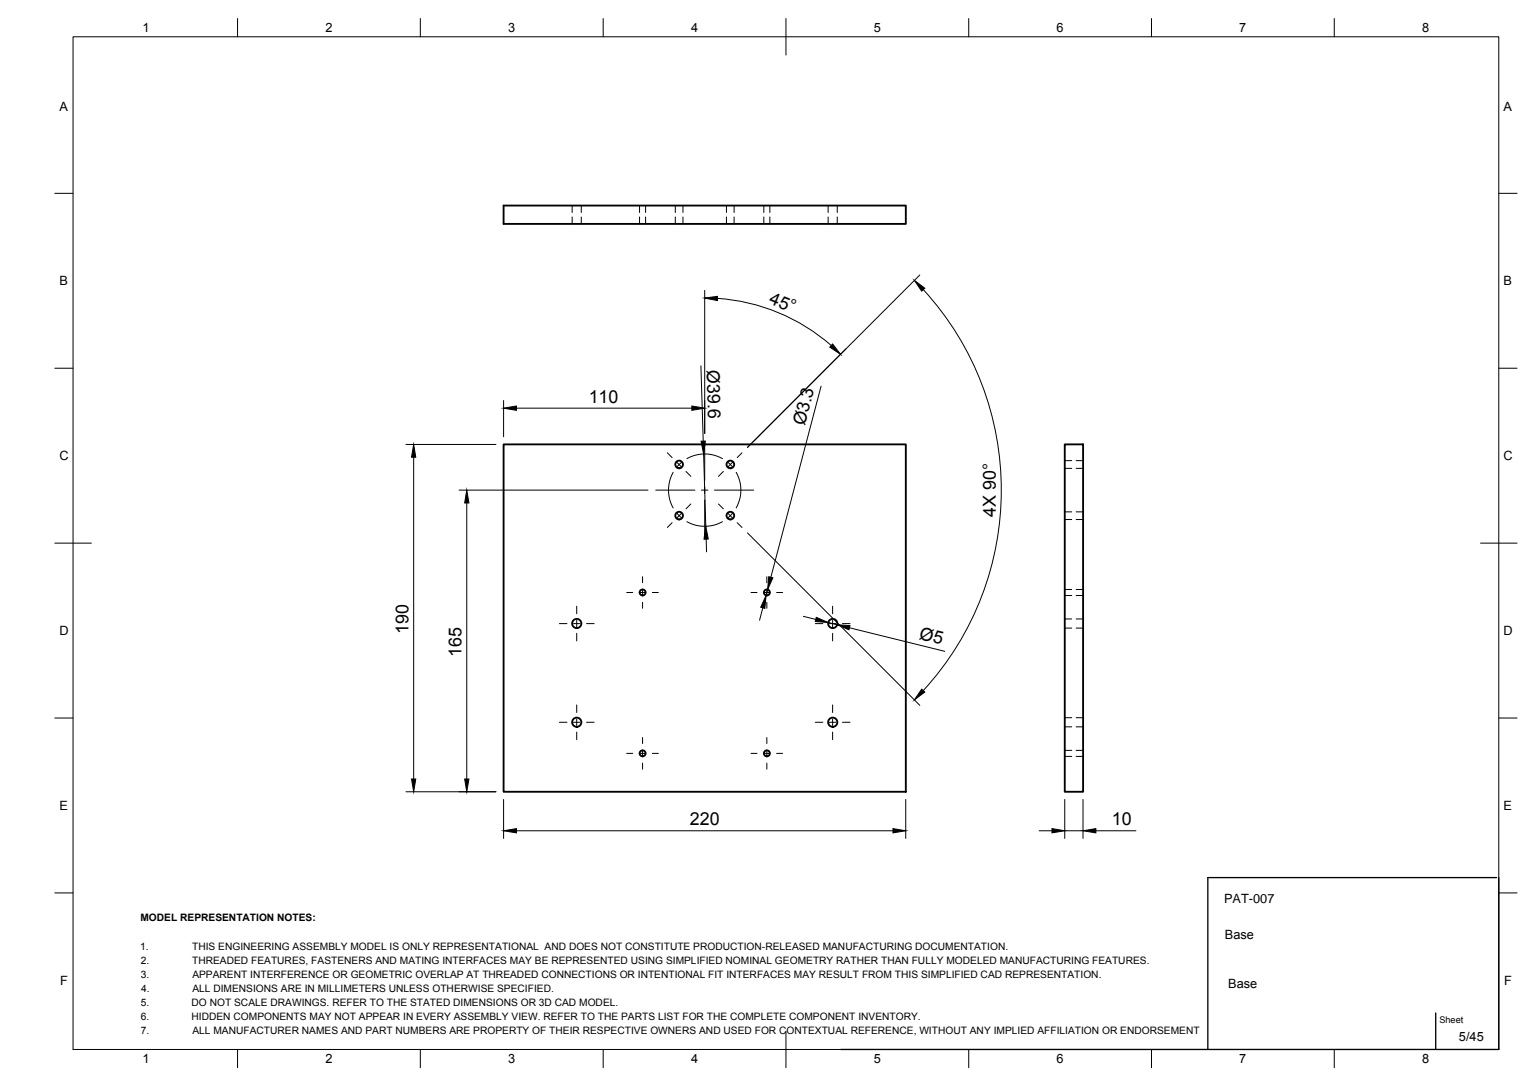
ISO-10303-21;
HEADER;
/* Generated by software containing ST-Developer
 * from STEP Tools, Inc. (www.steptools.com) 
 */

FILE_DESCRIPTION(
/* description */ ('Bearing friction torque test rig'),
/* implementation_level */ '2;1');

FILE_NAME(
/* name */ 'Base.step',
/* time_stamp */ '2026-10-28T03:24:04-07:00',
/* author */ (''),
/* organization */ (''),
/* preprocessor_version */ 'ST-DEVELOPER v20.2',
/* originating_system */ 'Autodesk Translation Framework v15.17.0.0',
/* authorisation */ '');

FILE_SCHEMA (('AUTOMOTIVE_DESIGN { 1 0 10303 214 3 1 1 }'));
ENDSEC;

DATA;
#10=MECHANICAL_DESIGN_GEOMETRIC_PRESENTATION_REPRESENTATION('',(#539),#14822);
#461=SHAPE_REPRESENTATION_RELATIONSHIP('SRR','None',#15000,#500);
#500=ADVANCED_BREP_SHAPE_REPRESENTATION('',(#593),#14780);
#539=STYLED_ITEM('',(#15263),#593);
#593=MANIFOLD_SOLID_BREP('Body1',#7655);
#644=FACE_BOUND('',#1561,.T.);
#645=FACE_BOUND('',#1562,.T.);
#646=FACE_BOUND('',#1563,.T.);
#647=FACE_BOUND('',#1564,.T.);
#648=FACE_BOUND('',#1565,.T.);
#649=FACE_BOUND('',#1566,.T.);
#650=FACE_BOUND('',#1567,.T.);
#651=FACE_BOUND('',#1568,.T.);
#652=FACE_BOUND('',#1569,.T.);
#653=FACE_BOUND('',#1570,.T.);
#654=FACE_BOUND('',#1571,.T.);
#655=FACE_BOUND('',#1572,.T.);
#656=FACE_BOUND('',#1574,.T.);
#657=FACE_BOUND('',#1575,.T.);
#658=FACE_BOUND('',#1576,.T.);
#659=FACE_BOUND('',#1577,.T.);
#660=FACE_BOUND('',#1578,.T.);
#661=FACE_BOUND('',#1579,.T.);
#662=FACE_BOUND('',#1580,.T.);
#663=FACE_BOUND('',#1581,.T.);
#664=FACE_BOUND('',#1582,.T.);
#665=FACE_BOUND('',#1583,.T.);
#666=FACE_BOUND('',#1584,.T.);
#667=FACE_BOUND('',#1585,.T.);
#874=PLANE('',#8181);
#875=PLANE('',#8182);
#876=PLANE('',#8183);
#877=PLANE('',#8184);
#878=PLANE('',#8185);
#879=PLANE('',#8186);
#1099=FACE_OUTER_BOUND('',#1544,.T.);
#1100=FACE_OUTER_BOUND('',#1545,.T.);
#1101=FACE_OUTER_BOUND('',#1546,.T.);
#1102=FACE_OUTER_BOUND('',#1547,.T.);
#1103=FACE_OUTER_BOUND('',#1548,.T.);
#1104=FACE_OUTER_BOUND('',#1549,.T.);
#1105=FACE_OUTER_BOUND('',#1550,.T.);
#1106=FACE_OUTER_BOUND('',#1551,.T.);
#1107=FACE_OUTER_BOUND('',#1552,.T.);
#1108=FACE_OUTER_BOUND('',#1553,.T.);
#1109=FACE_OUTER_BOUND('',#1554,.T.);
#1110=FACE_OUTER_BOUND('',#1555,.T.);
#1111=FACE_OUTER_BOUND('',#1556,.T.);
#1112=FACE_OUTER_BOUND('',#1557,.T.);
#1113=FACE_OUTER_BOUND('',#1558,.T.);
#1114=FACE_OUTER_BOUND('',#1559,.T.);
#1115=FACE_OUTER_BOUND('',#1560,.T.);
#1116=FACE_OUTER_BOUND('',#1573,.T.);
#1544=EDGE_LOOP('',(#5148,#5149,#5150,#5151));
#1545=EDGE_LOOP('',(#5152,#5153,#5154,#5155));
#1546=EDGE_LOOP('',(#5156,#5157,#5158,#5159));
#1547=EDGE_LOOP('',(#5160,#5161,#5162,#5163));
#1548=EDGE_LOOP('',(#5164,#5165,#5166,#5167));
#1549=EDGE_LOOP('',(#5168,#5169,#5170,#5171));
#1550=EDGE_LOOP('',(#5172,#5173,#5174,#5175));
#1551=EDGE_LOOP('',(#5176,#5177,#5178,#5179));
#1552=EDGE_LOOP('',(#5180,#5181,#5182,#5183));
#1553=EDGE_LOOP('',(#5184,#5185,#5186,#5187));
#1554=EDGE_LOOP('',(#5188,#5189,#5190,#5191));
#1555=EDGE_LOOP('',(#5192,#5193,#5194,#5195));
#1556=EDGE_LOOP('',(#5196,#5197,#5198,#5199));
#1557=EDGE_LOOP('',(#5200,#5201,#5202,#5203));
#1558=EDGE_LOOP('',(#5204,#5205,#5206,#5207));
#1559=EDGE_LOOP('',(#5208,#5209,#5210,#5211));
#1560=EDGE_LOOP('',(#5212,#5213,#5214,#5215));
#1561=EDGE_LOOP('',(#5216));
#1562=EDGE_LOOP('',(#5217));
#1563=EDGE_LOOP('',(#5218));
#1564=EDGE_LOOP('',(#5219));
#1565=EDGE_LOOP('',(#5220));
#1566=EDGE_LOOP('',(#5221));
#1567=EDGE_LOOP('',(#5222));
#1568=EDGE_LOOP('',(#5223));
#1569=EDGE_LOOP('',(#5224));
#1570=EDGE_LOOP('',(#5225));
#1571=EDGE_LOOP('',(#5226));
#1572=EDGE_LOOP('',(#5227));
#1573=EDGE_LOOP('',(#5228,#5229,#5230,#5231));
#1574=EDGE_LOOP('',(#5232));
#1575=EDGE_LOOP('',(#5233));
#1576=EDGE_LOOP('',(#5234));
#1577=EDGE_LOOP('',(#5235));
#1578=EDGE_LOOP('',(#5236));
#1579=EDGE_LOOP('',(#5237));
#1580=EDGE_LOOP('',(#5238));
#1581=EDGE_LOOP('',(#5239));
#1582=EDGE_LOOP('',(#5240));
#1583=EDGE_LOOP('',(#5241));
#1584=EDGE_LOOP('',(#5242));
#1585=EDGE_LOOP('',(#5243));
#2219=LINE('',#11665,#2663);
#2220=LINE('',#11671,#2664);
#2221=LINE('',#11677,#2665);
#2222=LINE('',#11683,#2666);
#2223=LINE('',#11689,#2667);
#2224=LINE('',#11695,#2668);
#2225=LINE('',#11701,#2669);
#2226=LINE('',#11707,#2670);
#2227=LINE('',#11713,#2671);
#2228=LINE('',#11719,#2672);
#2229=LINE('',#11725,#2673);
#2230=LINE('',#11731,#2674);
#2231=LINE('',#11736,#2675);
#2232=LINE('',#11738,#2676);
#2233=LINE('',#11740,#2677);
#2234=LINE('',#11741,#2678);
#2235=LINE('',#11744,#2679);
#2236=LINE('',#11746,#2680);
#2237=LINE('',#11747,#2681);
#2238=LINE('',#11750,#2682);
#2239=LINE('',#11752,#2683);
#2240=LINE('',#11753,#2684);
#2241=LINE('',#11755,#2685);
#2242=LINE('',#11756,#2686);
#2663=VECTOR('',#9176,0.165);
#2664=VECTOR('',#9183,0.165);
#2665=VECTOR('',#9190,0.165);
#2666=VECTOR('',#9197,0.165);
#2667=VECTOR('',#9204,0.210000000000001);
#2668=VECTOR('',#9211,0.210000000000001);
#2669=VECTOR('',#9218,0.210000000000001);
#2670=VECTOR('',#9225,0.210000000000001);
#2671=VECTOR('',#9232,0.25);
#2672=VECTOR('',#9239,0.25);
#2673=VECTOR('',#9246,0.25);
#2674=VECTOR('',#9253,0.25);
#2675=VECTOR('',#9258,1.);
#2676=VECTOR('',#9259,1.);
#2677=VECTOR('',#9260,1.);
#2678=VECTOR('',#9261,1.);
#2679=VECTOR('',#9264,1.);
#2680=VECTOR('',#9265,1.);
#2681=VECTOR('',#9266,1.);
#2682=VECTOR('',#9269,1.);
#2683=VECTOR('',#9270,1.);
#2684=VECTOR('',#9271,1.);
#2685=VECTOR('',#9274,1.);
#2686=VECTOR('',#9275,1.);
#3107=CIRCLE('',#8146,0.165);
#3108=CIRCLE('',#8147,0.165);
#3109=CIRCLE('',#8149,0.165);
#3110=CIRCLE('',#8150,0.165);
#3111=CIRCLE('',#8152,0.165);
#3112=CIRCLE('',#8153,0.165);
#3113=CIRCLE('',#8155,0.165);
#3114=CIRCLE('',#8156,0.165);
#3115=CIRCLE('',#8158,0.210000000000001);
#3116=CIRCLE('',#8159,0.210000000000001);
#3117=CIRCLE('',#8161,0.210000000000001);
#3118=CIRCLE('',#8162,0.210000000000001);
#3119=CIRCLE('',#8164,0.210000000000001);
#3120=CIRCLE('',#8165,0.210000000000001);
#3121=CIRCLE('',#8167,0.210000000000001);
#3122=CIRCLE('',#8168,0.210000000000001);
#3123=CIRCLE('',#8170,0.25);
#3124=CIRCLE('',#8171,0.25);
#3125=CIRCLE('',#8173,0.25);
#3126=CIRCLE('',#8174,0.25);
#3127=CIRCLE('',#8176,0.25);
#3128=CIRCLE('',#8177,0.25);
#3129=CIRCLE('',#8179,0.25);
#3130=CIRCLE('',#8180,0.25);
#3553=VERTEX_POINT('',#11662);
#3554=VERTEX_POINT('',#11664);
#3555=VERTEX_POINT('',#11668);
#3556=VERTEX_POINT('',#11670);
#3557=VERTEX_POINT('',#11674);
#3558=VERTEX_POINT('',#11676);
#3559=VERTEX_POINT('',#11680);
#3560=VERTEX_POINT('',#11682);
#3561=VERTEX_POINT('',#11686);
#3562=VERTEX_POINT('',#11688);
#3563=VERTEX_POINT('',#11692);
#3564=VERTEX_POINT('',#11694);
#3565=VERTEX_POINT('',#11698);
#3566=VERTEX_POINT('',#11700);
#3567=VERTEX_POINT('',#11704);
#3568=VERTEX_POINT('',#11706);
#3569=VERTEX_POINT('',#11710);
#3570=VERTEX_POINT('',#11712);
#3571=VERTEX_POINT('',#11716);
#3572=VERTEX_POINT('',#11718);
#3573=VERTEX_POINT('',#11722);
#3574=VERTEX_POINT('',#11724);
#3575=VERTEX_POINT('',#11728);
#3576=VERTEX_POINT('',#11730);
#3577=VERTEX_POINT('',#11734);
#3578=VERTEX_POINT('',#11735);
#3579=VERTEX_POINT('',#11737);
#3580=VERTEX_POINT('',#11739);
#3581=VERTEX_POINT('',#11743);
#3582=VERTEX_POINT('',#11745);
#3583=VERTEX_POINT('',#11749);
#3584=VERTEX_POINT('',#11751);
#4200=EDGE_CURVE('',#3553,#3553,#3107,.T.);
#4201=EDGE_CURVE('',#3553,#3554,#2219,.T.);
#4202=EDGE_CURVE('',#3554,#3554,#3108,.T.);
#4203=EDGE_CURVE('',#3555,#3555,#3109,.T.);
#4204=EDGE_CURVE('',#3555,#3556,#2220,.T.);
#4205=EDGE_CURVE('',#3556,#3556,#3110,.T.);
#4206=EDGE_CURVE('',#3557,#3557,#3111,.T.);
#4207=EDGE_CURVE('',#3557,#3558,#2221,.T.);
#4208=EDGE_CURVE('',#3558,#3558,#3112,.T.);
#4209=EDGE_CURVE('',#3559,#3559,#3113,.T.);
#4210=EDGE_CURVE('',#3559,#3560,#2222,.T.);
#4211=EDGE_CURVE('',#3560,#3560,#3114,.T.);
#4212=EDGE_CURVE('',#3561,#3561,#3115,.T.);
#4213=EDGE_CURVE('',#3561,#3562,#2223,.T.);
#4214=EDGE_CURVE('',#3562,#3562,#3116,.T.);
#4215=EDGE_CURVE('',#3563,#3563,#3117,.T.);
#4216=EDGE_CURVE('',#3563,#3564,#2224,.T.);
#4217=EDGE_CURVE('',#3564,#3564,#3118,.T.);
#4218=EDGE_CURVE('',#3565,#3565,#3119,.T.);
#4219=EDGE_CURVE('',#3565,#3566,#2225,.T.);
#4220=EDGE_CURVE('',#3566,#3566,#3120,.T.);
#4221=EDGE_CURVE('',#3567,#3567,#3121,.T.);
#4222=EDGE_CURVE('',#3567,#3568,#2226,.T.);
#4223=EDGE_CURVE('',#3568,#3568,#3122,.T.);
#4224=EDGE_CURVE('',#3569,#3569,#3123,.T.);
#4225=EDGE_CURVE('',#3569,#3570,#2227,.T.);
#4226=EDGE_CURVE('',#3570,#3570,#3124,.T.);
#4227=EDGE_CURVE('',#3571,#3571,#3125,.T.);
#4228=EDGE_CURVE('',#3571,#3572,#2228,.T.);
#4229=EDGE_CURVE('',#3572,#3572,#3126,.T.);
#4230=EDGE_CURVE('',#3573,#3573,#3127,.T.);
#4231=EDGE_CURVE('',#3573,#3574,#2229,.T.);
#4232=EDGE_CURVE('',#3574,#3574,#3128,.T.);
#4233=EDGE_CURVE('',#3575,#3575,#3129,.T.);
#4234=EDGE_CURVE('',#3575,#3576,#2230,.T.);
#4235=EDGE_CURVE('',#3576,#3576,#3130,.T.);
#4236=EDGE_CURVE('',#3577,#3578,#2231,.T.);
#4237=EDGE_CURVE('',#3578,#3579,#2232,.T.);
#4238=EDGE_CURVE('',#3580,#3579,#2233,.T.);
#4239=EDGE_CURVE('',#3577,#3580,#2234,.T.);
#4240=EDGE_CURVE('',#3581,#3577,#2235,.T.);
#4241=EDGE_CURVE('',#3582,#3580,#2236,.T.);
#4242=EDGE_CURVE('',#3581,#3582,#2237,.T.);
#4243=EDGE_CURVE('',#3583,#3581,#2238,.T.);
#4244=EDGE_CURVE('',#3584,#3582,#2239,.T.);
#4245=EDGE_CURVE('',#3583,#3584,#2240,.T.);
#4246=EDGE_CURVE('',#3578,#3583,#2241,.T.);
#4247=EDGE_CURVE('',#3579,#3584,#2242,.T.);
#5148=ORIENTED_EDGE('',*,*,#4200,.F.);
#5149=ORIENTED_EDGE('',*,*,#4201,.T.);
#5150=ORIENTED_EDGE('',*,*,#4202,.F.);
#5151=ORIENTED_EDGE('',*,*,#4201,.F.);
#5152=ORIENTED_EDGE('',*,*,#4203,.F.);
#5153=ORIENTED_EDGE('',*,*,#4204,.T.);
#5154=ORIENTED_EDGE('',*,*,#4205,.F.);
#5155=ORIENTED_EDGE('',*,*,#4204,.F.);
#5156=ORIENTED_EDGE('',*,*,#4206,.F.);
#5157=ORIENTED_EDGE('',*,*,#4207,.T.);
#5158=ORIENTED_EDGE('',*,*,#4208,.F.);
#5159=ORIENTED_EDGE('',*,*,#4207,.F.);
#5160=ORIENTED_EDGE('',*,*,#4209,.F.);
#5161=ORIENTED_EDGE('',*,*,#4210,.T.);
#5162=ORIENTED_EDGE('',*,*,#4211,.F.);
#5163=ORIENTED_EDGE('',*,*,#4210,.F.);
#5164=ORIENTED_EDGE('',*,*,#4212,.F.);
#5165=ORIENTED_EDGE('',*,*,#4213,.T.);
#5166=ORIENTED_EDGE('',*,*,#4214,.F.);
#5167=ORIENTED_EDGE('',*,*,#4213,.F.);
#5168=ORIENTED_EDGE('',*,*,#4215,.F.);
#5169=ORIENTED_EDGE('',*,*,#4216,.T.);
#5170=ORIENTED_EDGE('',*,*,#4217,.F.);
#5171=ORIENTED_EDGE('',*,*,#4216,.F.);
#5172=ORIENTED_EDGE('',*,*,#4218,.F.);
#5173=ORIENTED_EDGE('',*,*,#4219,.T.);
#5174=ORIENTED_EDGE('',*,*,#4220,.F.);
#5175=ORIENTED_EDGE('',*,*,#4219,.F.);
#5176=ORIENTED_EDGE('',*,*,#4221,.F.);
#5177=ORIENTED_EDGE('',*,*,#4222,.T.);
#5178=ORIENTED_EDGE('',*,*,#4223,.F.);
#5179=ORIENTED_EDGE('',*,*,#4222,.F.);
#5180=ORIENTED_EDGE('',*,*,#4224,.F.);
#5181=ORIENTED_EDGE('',*,*,#4225,.T.);
#5182=ORIENTED_EDGE('',*,*,#4226,.F.);
#5183=ORIENTED_EDGE('',*,*,#4225,.F.);
#5184=ORIENTED_EDGE('',*,*,#4227,.F.);
#5185=ORIENTED_EDGE('',*,*,#4228,.T.);
#5186=ORIENTED_EDGE('',*,*,#4229,.F.);
#5187=ORIENTED_EDGE('',*,*,#4228,.F.);
#5188=ORIENTED_EDGE('',*,*,#4230,.F.);
#5189=ORIENTED_EDGE('',*,*,#4231,.T.);
#5190=ORIENTED_EDGE('',*,*,#4232,.F.);
#5191=ORIENTED_EDGE('',*,*,#4231,.F.);
#5192=ORIENTED_EDGE('',*,*,#4233,.F.);
#5193=ORIENTED_EDGE('',*,*,#4234,.T.);
#5194=ORIENTED_EDGE('',*,*,#4235,.F.);
#5195=ORIENTED_EDGE('',*,*,#4234,.F.);
#5196=ORIENTED_EDGE('',*,*,#4236,.T.);
#5197=ORIENTED_EDGE('',*,*,#4237,.T.);
#5198=ORIENTED_EDGE('',*,*,#4238,.F.);
#5199=ORIENTED_EDGE('',*,*,#4239,.F.);
#5200=ORIENTED_EDGE('',*,*,#4240,.T.);
#5201=ORIENTED_EDGE('',*,*,#4239,.T.);
#5202=ORIENTED_EDGE('',*,*,#4241,.F.);
#5203=ORIENTED_EDGE('',*,*,#4242,.F.);
#5204=ORIENTED_EDGE('',*,*,#4243,.T.);
#5205=ORIENTED_EDGE('',*,*,#4242,.T.);
#5206=ORIENTED_EDGE('',*,*,#4244,.F.);
#5207=ORIENTED_EDGE('',*,*,#4245,.F.);
#5208=ORIENTED_EDGE('',*,*,#4246,.T.);
#5209=ORIENTED_EDGE('',*,*,#4245,.T.);
#5210=ORIENTED_EDGE('',*,*,#4247,.F.);
#5211=ORIENTED_EDGE('',*,*,#4237,.F.);
#5212=ORIENTED_EDGE('',*,*,#4247,.T.);
#5213=ORIENTED_EDGE('',*,*,#4244,.T.);
#5214=ORIENTED_EDGE('',*,*,#4241,.T.);
#5215=ORIENTED_EDGE('',*,*,#4238,.T.);
#5216=ORIENTED_EDGE('',*,*,#4205,.T.);
#5217=ORIENTED_EDGE('',*,*,#4211,.T.);
#5218=ORIENTED_EDGE('',*,*,#4235,.T.);
#5219=ORIENTED_EDGE('',*,*,#4232,.T.);
#5220=ORIENTED_EDGE('',*,*,#4229,.T.);
#5221=ORIENTED_EDGE('',*,*,#4226,.T.);
#5222=ORIENTED_EDGE('',*,*,#4223,.T.);
#5223=ORIENTED_EDGE('',*,*,#4220,.T.);
#5224=ORIENTED_EDGE('',*,*,#4217,.T.);
#5225=ORIENTED_EDGE('',*,*,#4214,.T.);
#5226=ORIENTED_EDGE('',*,*,#4208,.T.);
#5227=ORIENTED_EDGE('',*,*,#4202,.T.);
#5228=ORIENTED_EDGE('',*,*,#4246,.F.);
#5229=ORIENTED_EDGE('',*,*,#4236,.F.);
#5230=ORIENTED_EDGE('',*,*,#4240,.F.);
#5231=ORIENTED_EDGE('',*,*,#4243,.F.);
#5232=ORIENTED_EDGE('',*,*,#4203,.T.);
#5233=ORIENTED_EDGE('',*,*,#4209,.T.);
#5234=ORIENTED_EDGE('',*,*,#4233,.T.);
#5235=ORIENTED_EDGE('',*,*,#4230,.T.);
#5236=ORIENTED_EDGE('',*,*,#4227,.T.);
#5237=ORIENTED_EDGE('',*,*,#4224,.T.);
#5238=ORIENTED_EDGE('',*,*,#4221,.T.);
#5239=ORIENTED_EDGE('',*,*,#4218,.T.);
#5240=ORIENTED_EDGE('',*,*,#4215,.T.);
#5241=ORIENTED_EDGE('',*,*,#4212,.T.);
#5242=ORIENTED_EDGE('',*,*,#4206,.T.);
#5243=ORIENTED_EDGE('',*,*,#4200,.T.);
#7044=CYLINDRICAL_SURFACE('',#8145,0.165);
#7045=CYLINDRICAL_SURFACE('',#8148,0.165);
#7046=CYLINDRICAL_SURFACE('',#8151,0.165);
#7047=CYLINDRICAL_SURFACE('',#8154,0.165);
#7048=CYLINDRICAL_SURFACE('',#8157,0.210000000000001);
#7049=CYLINDRICAL_SURFACE('',#8160,0.210000000000001);
#7050=CYLINDRICAL_SURFACE('',#8163,0.210000000000001);
#7051=CYLINDRICAL_SURFACE('',#8166,0.210000000000001);
#7052=CYLINDRICAL_SURFACE('',#8169,0.25);
#7053=CYLINDRICAL_SURFACE('',#8172,0.25);
#7054=CYLINDRICAL_SURFACE('',#8175,0.25);
#7055=CYLINDRICAL_SURFACE('',#8178,0.25);
#7210=ADVANCED_FACE('',(#1099),#7044,.F.);
#7211=ADVANCED_FACE('',(#1100),#7045,.F.);
#7212=ADVANCED_FACE('',(#1101),#7046,.F.);
#7213=ADVANCED_FACE('',(#1102),#7047,.F.);
#7214=ADVANCED_FACE('',(#1103),#7048,.F.);
#7215=ADVANCED_FACE('',(#1104),#7049,.F.);
#7216=ADVANCED_FACE('',(#1105),#7050,.F.);
#7217=ADVANCED_FACE('',(#1106),#7051,.F.);
#7218=ADVANCED_FACE('',(#1107),#7052,.F.);
#7219=ADVANCED_FACE('',(#1108),#7053,.F.);
#7220=ADVANCED_FACE('',(#1109),#7054,.F.);
#7221=ADVANCED_FACE('',(#1110),#7055,.F.);
#7222=ADVANCED_FACE('',(#1111),#874,.T.);
#7223=ADVANCED_FACE('',(#1112),#875,.T.);
#7224=ADVANCED_FACE('',(#1113),#876,.T.);
#7225=ADVANCED_FACE('',(#1114),#877,.T.);
#7226=ADVANCED_FACE('',(#1115,#644,#645,#646,#647,#648,#649,#650,#651,#652,
#653,#654,#655),#878,.T.);
#7227=ADVANCED_FACE('',(#1116,#656,#657,#658,#659,#660,#661,#662,#663,#664,
#665,#666,#667),#879,.F.);
#7655=CLOSED_SHELL('',(#7210,#7211,#7212,#7213,#7214,#7215,#7216,#7217,
#7218,#7219,#7220,#7221,#7222,#7223,#7224,#7225,#7226,#7227));
#8144=AXIS2_PLACEMENT_3D('',#11660,#9170,#9171);
#8145=AXIS2_PLACEMENT_3D('',#11661,#9172,#9173);
#8146=AXIS2_PLACEMENT_3D('',#11663,#9174,#9175);
#8147=AXIS2_PLACEMENT_3D('',#11666,#9177,#9178);
#8148=AXIS2_PLACEMENT_3D('',#11667,#9179,#9180);
#8149=AXIS2_PLACEMENT_3D('',#11669,#9181,#9182);
#8150=AXIS2_PLACEMENT_3D('',#11672,#9184,#9185);
#8151=AXIS2_PLACEMENT_3D('',#11673,#9186,#9187);
#8152=AXIS2_PLACEMENT_3D('',#11675,#9188,#9189);
#8153=AXIS2_PLACEMENT_3D('',#11678,#9191,#9192);
#8154=AXIS2_PLACEMENT_3D('',#11679,#9193,#9194);
#8155=AXIS2_PLACEMENT_3D('',#11681,#9195,#9196);
#8156=AXIS2_PLACEMENT_3D('',#11684,#9198,#9199);
#8157=AXIS2_PLACEMENT_3D('',#11685,#9200,#9201);
#8158=AXIS2_PLACEMENT_3D('',#11687,#9202,#9203);
#8159=AXIS2_PLACEMENT_3D('',#11690,#9205,#9206);
#8160=AXIS2_PLACEMENT_3D('',#11691,#9207,#9208);
#8161=AXIS2_PLACEMENT_3D('',#11693,#9209,#9210);
#8162=AXIS2_PLACEMENT_3D('',#11696,#9212,#9213);
#8163=AXIS2_PLACEMENT_3D('',#11697,#9214,#9215);
#8164=AXIS2_PLACEMENT_3D('',#11699,#9216,#9217);
#8165=AXIS2_PLACEMENT_3D('',#11702,#9219,#9220);
#8166=AXIS2_PLACEMENT_3D('',#11703,#9221,#9222);
#8167=AXIS2_PLACEMENT_3D('',#11705,#9223,#9224);
#8168=AXIS2_PLACEMENT_3D('',#11708,#9226,#9227);
#8169=AXIS2_PLACEMENT_3D('',#11709,#9228,#9229);
#8170=AXIS2_PLACEMENT_3D('',#11711,#9230,#9231);
#8171=AXIS2_PLACEMENT_3D('',#11714,#9233,#9234);
#8172=AXIS2_PLACEMENT_3D('',#11715,#9235,#9236);
#8173=AXIS2_PLACEMENT_3D('',#11717,#9237,#9238);
#8174=AXIS2_PLACEMENT_3D('',#11720,#9240,#9241);
#8175=AXIS2_PLACEMENT_3D('',#11721,#9242,#9243);
#8176=AXIS2_PLACEMENT_3D('',#11723,#9244,#9245);
#8177=AXIS2_PLACEMENT_3D('',#11726,#9247,#9248);
#8178=AXIS2_PLACEMENT_3D('',#11727,#9249,#9250);
#8179=AXIS2_PLACEMENT_3D('',#11729,#9251,#9252);
#8180=AXIS2_PLACEMENT_3D('',#11732,#9254,#9255);
#8181=AXIS2_PLACEMENT_3D('',#11733,#9256,#9257);
#8182=AXIS2_PLACEMENT_3D('',#11742,#9262,#9263);
#8183=AXIS2_PLACEMENT_3D('',#11748,#9267,#9268);
#8184=AXIS2_PLACEMENT_3D('',#11754,#9272,#9273);
#8185=AXIS2_PLACEMENT_3D('',#11757,#9276,#9277);
#8186=AXIS2_PLACEMENT_3D('',#11758,#9278,#9279);
#9170=DIRECTION('axis',(0.,0.,1.));
#9171=DIRECTION('refdir',(1.,0.,0.));
#9172=DIRECTION('center_axis',(0.,0.,1.));
#9173=DIRECTION('ref_axis',(1.,0.,0.));
#9174=DIRECTION('center_axis',(0.,0.,1.));
#9175=DIRECTION('ref_axis',(1.,0.,0.));
#9176=DIRECTION('',(0.,0.,1.));
#9177=DIRECTION('center_axis',(0.,0.,-1.));
#9178=DIRECTION('ref_axis',(1.,0.,0.));
#9179=DIRECTION('center_axis',(0.,0.,1.));
#9180=DIRECTION('ref_axis',(1.,0.,0.));
#9181=DIRECTION('center_axis',(0.,0.,1.));
#9182=DIRECTION('ref_axis',(1.,0.,0.));
#9183=DIRECTION('',(0.,0.,1.));
#9184=DIRECTION('center_axis',(0.,0.,-1.));
#9185=DIRECTION('ref_axis',(1.,0.,0.));
#9186=DIRECTION('center_axis',(0.,0.,1.));
#9187=DIRECTION('ref_axis',(1.,0.,0.));
#9188=DIRECTION('center_axis',(0.,0.,1.));
#9189=DIRECTION('ref_axis',(1.,0.,0.));
#9190=DIRECTION('',(0.,0.,1.));
#9191=DIRECTION('center_axis',(0.,0.,-1.));
#9192=DIRECTION('ref_axis',(1.,0.,0.));
#9193=DIRECTION('center_axis',(0.,0.,1.));
#9194=DIRECTION('ref_axis',(1.,0.,0.));
#9195=DIRECTION('center_axis',(0.,0.,1.));
#9196=DIRECTION('ref_axis',(1.,0.,0.));
#9197=DIRECTION('',(0.,0.,1.));
#9198=DIRECTION('center_axis',(0.,0.,-1.));
#9199=DIRECTION('ref_axis',(1.,0.,0.));
#9200=DIRECTION('center_axis',(0.,0.,1.));
#9201=DIRECTION('ref_axis',(1.,0.,0.));
#9202=DIRECTION('center_axis',(0.,0.,1.));
#9203=DIRECTION('ref_axis',(1.,0.,0.));
#9204=DIRECTION('',(0.,0.,1.));
#9205=DIRECTION('center_axis',(0.,0.,-1.));
#9206=DIRECTION('ref_axis',(1.,0.,0.));
#9207=DIRECTION('center_axis',(0.,0.,1.));
#9208=DIRECTION('ref_axis',(1.,0.,0.));
#9209=DIRECTION('center_axis',(0.,0.,1.));
#9210=DIRECTION('ref_axis',(1.,0.,0.));
#9211=DIRECTION('',(0.,0.,1.));
#9212=DIRECTION('center_axis',(0.,0.,-1.));
#9213=DIRECTION('ref_axis',(1.,0.,0.));
#9214=DIRECTION('center_axis',(0.,0.,1.));
#9215=DIRECTION('ref_axis',(1.,0.,0.));
#9216=DIRECTION('center_axis',(0.,0.,1.));
#9217=DIRECTION('ref_axis',(1.,0.,0.));
#9218=DIRECTION('',(0.,0.,1.));
#9219=DIRECTION('center_axis',(0.,0.,-1.));
#9220=DIRECTION('ref_axis',(1.,0.,0.));
#9221=DIRECTION('center_axis',(0.,0.,1.));
#9222=DIRECTION('ref_axis',(1.,0.,0.));
#9223=DIRECTION('center_axis',(0.,0.,1.));
#9224=DIRECTION('ref_axis',(1.,0.,0.));
#9225=DIRECTION('',(0.,0.,1.));
#9226=DIRECTION('center_axis',(0.,0.,-1.));
#9227=DIRECTION('ref_axis',(1.,0.,0.));
#9228=DIRECTION('center_axis',(0.,0.,1.));
#9229=DIRECTION('ref_axis',(1.,0.,0.));
#9230=DIRECTION('center_axis',(0.,0.,1.));
#9231=DIRECTION('ref_axis',(1.,0.,0.));
#9232=DIRECTION('',(0.,0.,1.));
#9233=DIRECTION('center_axis',(0.,0.,-1.));
#9234=DIRECTION('ref_axis',(1.,0.,0.));
#9235=DIRECTION('center_axis',(0.,0.,1.));
#9236=DIRECTION('ref_axis',(1.,0.,0.));
#9237=DIRECTION('center_axis',(0.,0.,1.));
#9238=DIRECTION('ref_axis',(1.,0.,0.));
#9239=DIRECTION('',(0.,0.,1.));
#9240=DIRECTION('center_axis',(0.,0.,-1.));
#9241=DIRECTION('ref_axis',(1.,0.,0.));
#9242=DIRECTION('center_axis',(0.,0.,1.));
#9243=DIRECTION('ref_axis',(1.,0.,0.));
#9244=DIRECTION('center_axis',(0.,0.,1.));
#9245=DIRECTION('ref_axis',(1.,0.,0.));
#9246=DIRECTION('',(0.,0.,1.));
#9247=DIRECTION('center_axis',(0.,0.,-1.));
#9248=DIRECTION('ref_axis',(1.,0.,0.));
#9249=DIRECTION('center_axis',(0.,0.,1.));
#9250=DIRECTION('ref_axis',(1.,0.,0.));
#9251=DIRECTION('center_axis',(0.,0.,1.));
#9252=DIRECTION('ref_axis',(1.,0.,0.));
#9253=DIRECTION('',(0.,0.,1.));
#9254=DIRECTION('center_axis',(0.,0.,-1.));
#9255=DIRECTION('ref_axis',(1.,0.,0.));
#9256=DIRECTION('center_axis',(0.,1.,0.));
#9257=DIRECTION('ref_axis',(-1.,0.,0.));
#9258=DIRECTION('',(-1.,0.,0.));
#9259=DIRECTION('',(0.,0.,1.));
#9260=DIRECTION('',(-1.,0.,0.));
#9261=DIRECTION('',(0.,0.,1.));
#9262=DIRECTION('center_axis',(1.,0.,0.));
#9263=DIRECTION('ref_axis',(0.,1.,0.));
#9264=DIRECTION('',(0.,1.,0.));
#9265=DIRECTION('',(0.,1.,0.));
#9266=DIRECTION('',(0.,0.,1.));
#9267=DIRECTION('center_axis',(0.,-1.,0.));
#9268=DIRECTION('ref_axis',(1.,0.,0.));
#9269=DIRECTION('',(1.,0.,0.));
#9270=DIRECTION('',(1.,0.,0.));
#9271=DIRECTION('',(0.,0.,1.));
#9272=DIRECTION('center_axis',(-1.,0.,0.));
#9273=DIRECTION('ref_axis',(0.,-1.,0.));
#9274=DIRECTION('',(0.,-1.,0.));
#9275=DIRECTION('',(0.,-1.,0.));
#9276=DIRECTION('center_axis',(0.,0.,1.));
#9277=DIRECTION('ref_axis',(1.,0.,0.));
#9278=DIRECTION('center_axis',(0.,0.,1.));
#9279=DIRECTION('ref_axis',(1.,0.,0.));
#11660=CARTESIAN_POINT('',(0.,0.,0.));
#11661=CARTESIAN_POINT('Origin',(4.4,3.4,-0.1));
#11662=CARTESIAN_POINT('',(4.235,3.4,0.));
#11663=CARTESIAN_POINT('Origin',(4.4,3.4,0.));
#11664=CARTESIAN_POINT('',(4.235,3.4,1.));
#11665=CARTESIAN_POINT('',(4.235,3.4,-0.1));
#11666=CARTESIAN_POINT('Origin',(4.4,3.4,1.));
#11667=CARTESIAN_POINT('Origin',(4.4,-3.4,-0.1));
#11668=CARTESIAN_POINT('',(4.235,-3.4,0.));
#11669=CARTESIAN_POINT('Origin',(4.4,-3.4,0.));
#11670=CARTESIAN_POINT('',(4.235,-3.4,1.));
#11671=CARTESIAN_POINT('',(4.235,-3.4,-0.1));
#11672=CARTESIAN_POINT('Origin',(4.4,-3.4,1.));
#11673=CARTESIAN_POINT('Origin',(-4.4,3.4,-0.1));
#11674=CARTESIAN_POINT('',(-4.565,3.4,0.));
#11675=CARTESIAN_POINT('Origin',(-4.4,3.4,0.));
#11676=CARTESIAN_POINT('',(-4.565,3.4,1.));
#11677=CARTESIAN_POINT('',(-4.565,3.4,-0.1));
#11678=CARTESIAN_POINT('Origin',(-4.4,3.4,1.));
#11679=CARTESIAN_POINT('Origin',(-4.4,-3.4,-0.1));
#11680=CARTESIAN_POINT('',(-4.565,-3.4,0.));
#11681=CARTESIAN_POINT('Origin',(-4.4,-3.4,0.));
#11682=CARTESIAN_POINT('',(-4.565,-3.4,1.));
#11683=CARTESIAN_POINT('',(-4.565,-3.4,-0.1));
#11684=CARTESIAN_POINT('Origin',(-4.4,-3.4,1.));
#11685=CARTESIAN_POINT('Origin',(11.4,-1.4,-0.1));
#11686=CARTESIAN_POINT('',(11.19,-1.4,0.));
#11687=CARTESIAN_POINT('Origin',(11.4,-1.4,0.));
#11688=CARTESIAN_POINT('',(11.19,-1.4,1.));
#11689=CARTESIAN_POINT('',(11.19,-1.4,-0.1));
#11690=CARTESIAN_POINT('Origin',(11.4,-1.4,1.));
#11691=CARTESIAN_POINT('Origin',(8.6,1.4,-0.1));
#11692=CARTESIAN_POINT('',(8.39,1.4,0.));
#11693=CARTESIAN_POINT('Origin',(8.6,1.4,0.));
#11694=CARTESIAN_POINT('',(8.39,1.4,1.));
#11695=CARTESIAN_POINT('',(8.39,1.4,-0.1));
#11696=CARTESIAN_POINT('Origin',(8.6,1.4,1.));
#11697=CARTESIAN_POINT('Origin',(8.6,-1.4,-0.1));
#11698=CARTESIAN_POINT('',(8.39,-1.4,0.));
#11699=CARTESIAN_POINT('Origin',(8.6,-1.4,0.));
#11700=CARTESIAN_POINT('',(8.39,-1.4,1.));
#11701=CARTESIAN_POINT('',(8.39,-1.4,-0.1));
#11702=CARTESIAN_POINT('Origin',(8.6,-1.4,1.));
#11703=CARTESIAN_POINT('Origin',(11.4,1.4,-0.1));
#11704=CARTESIAN_POINT('',(11.19,1.4,0.));
#11705=CARTESIAN_POINT('Origin',(11.4,1.4,0.));
#11706=CARTESIAN_POINT('',(11.19,1.4,1.));
#11707=CARTESIAN_POINT('',(11.19,1.4,-0.1));
#11708=CARTESIAN_POINT('Origin',(11.4,1.4,1.));
#11709=CARTESIAN_POINT('Origin',(-2.7,7.,-0.1));
#11710=CARTESIAN_POINT('',(-2.95,7.,0.));
#11711=CARTESIAN_POINT('Origin',(-2.7,7.,0.));
#11712=CARTESIAN_POINT('',(-2.95,7.,1.));
#11713=CARTESIAN_POINT('',(-2.95,7.,-0.1));
#11714=CARTESIAN_POINT('Origin',(-2.7,7.,1.));
#11715=CARTESIAN_POINT('Origin',(2.7,7.,-0.1));
#11716=CARTESIAN_POINT('',(2.45,7.,0.));
#11717=CARTESIAN_POINT('Origin',(2.7,7.,0.));
#11718=CARTESIAN_POINT('',(2.45,7.,1.));
#11719=CARTESIAN_POINT('',(2.45,7.,-0.1));
#11720=CARTESIAN_POINT('Origin',(2.7,7.,1.));
#11721=CARTESIAN_POINT('Origin',(-2.7,-7.,-0.1));
#11722=CARTESIAN_POINT('',(-2.95,-7.,0.));
#11723=CARTESIAN_POINT('Origin',(-2.7,-7.,0.));
#11724=CARTESIAN_POINT('',(-2.95,-7.,1.));
#11725=CARTESIAN_POINT('',(-2.95,-7.,-0.1));
#11726=CARTESIAN_POINT('Origin',(-2.7,-7.,1.));
#11727=CARTESIAN_POINT('Origin',(2.7,-7.,-0.1));
#11728=CARTESIAN_POINT('',(2.45,-7.,0.));
#11729=CARTESIAN_POINT('Origin',(2.7,-7.,0.));
#11730=CARTESIAN_POINT('',(2.45,-7.,1.));
#11731=CARTESIAN_POINT('',(2.45,-7.,-0.1));
#11732=CARTESIAN_POINT('Origin',(2.7,-7.,1.));
#11733=CARTESIAN_POINT('Origin',(12.5,11.,0.));
#11734=CARTESIAN_POINT('',(12.5,11.,0.));
#11735=CARTESIAN_POINT('',(-6.5,11.,0.));
#11736=CARTESIAN_POINT('',(12.5,11.,0.));
#11737=CARTESIAN_POINT('',(-6.5,11.,1.));
#11738=CARTESIAN_POINT('',(-6.5,11.,0.));
#11739=CARTESIAN_POINT('',(12.5,11.,1.));
#11740=CARTESIAN_POINT('',(12.5,11.,1.));
#11741=CARTESIAN_POINT('',(12.5,11.,0.));
#11742=CARTESIAN_POINT('Origin',(12.5,-11.,0.));
#11743=CARTESIAN_POINT('',(12.5,-11.,0.));
#11744=CARTESIAN_POINT('',(12.5,-11.,0.));
#11745=CARTESIAN_POINT('',(12.5,-11.,1.));
#11746=CARTESIAN_POINT('',(12.5,-11.,1.));
#11747=CARTESIAN_POINT('',(12.5,-11.,0.));
#11748=CARTESIAN_POINT('Origin',(-6.5,-11.,0.));
#11749=CARTESIAN_POINT('',(-6.5,-11.,0.));
#11750=CARTESIAN_POINT('',(-6.5,-11.,0.));
#11751=CARTESIAN_POINT('',(-6.5,-11.,1.));
#11752=CARTESIAN_POINT('',(-6.5,-11.,1.));
#11753=CARTESIAN_POINT('',(-6.5,-11.,0.));
#11754=CARTESIAN_POINT('Origin',(-6.5,11.,0.));
#11755=CARTESIAN_POINT('',(-6.5,11.,0.));
#11756=CARTESIAN_POINT('',(-6.5,11.,1.));
#11757=CARTESIAN_POINT('Origin',(3.,0.,1.));
#11758=CARTESIAN_POINT('Origin',(3.,0.,0.));
#14735=UNCERTAINTY_MEASURE_WITH_UNIT(LENGTH_MEASURE(0.001),#14823,
'DISTANCE_ACCURACY_VALUE',
'Maximum model space distance between geometric entities at asserted c
onnectivities');
#14777=UNCERTAINTY_MEASURE_WITH_UNIT(LENGTH_MEASURE(0.001),#14823,
'DISTANCE_ACCURACY_VALUE',
'Maximum model space distance between geometric entities at asserted c
onnectivities');
#14780=(
GEOMETRIC_REPRESENTATION_CONTEXT(3)
GLOBAL_UNCERTAINTY_ASSIGNED_CONTEXT((#14735))
GLOBAL_UNIT_ASSIGNED_CONTEXT((#14823,#14825,#14826))
REPRESENTATION_CONTEXT('','3D')
);
#14822=(
GEOMETRIC_REPRESENTATION_CONTEXT(3)
GLOBAL_UNCERTAINTY_ASSIGNED_CONTEXT((#14777))
GLOBAL_UNIT_ASSIGNED_CONTEXT((#14823,#14825,#14826))
REPRESENTATION_CONTEXT('','3D')
);
#14823=(
LENGTH_UNIT()
NAMED_UNIT(*)
SI_UNIT(.CENTI.,.METRE.)
);
#14825=(
NAMED_UNIT(*)
PLANE_ANGLE_UNIT()
SI_UNIT($,.RADIAN.)
);
#14826=(
NAMED_UNIT(*)
SI_UNIT($,.STERADIAN.)
SOLID_ANGLE_UNIT()
);
#14829=SHAPE_DEFINITION_REPRESENTATION(#14873,#15000);
#14873=PRODUCT_DEFINITION_SHAPE('',$,#15045);
#15000=SHAPE_REPRESENTATION('',(#8144),#14780);
#15042=PRODUCT_DEFINITION_CONTEXT('part definition',#15176,'design');
#15045=PRODUCT_DEFINITION('Base','Base',#15089,#15042);
#15089=PRODUCT_DEFINITION_FORMATION('',$,#15180);
#15176=APPLICATION_CONTEXT(
'Core Data for Automotive Mechanical Design Process');
#15177=PRODUCT_CONTEXT('part definition',#15176,'mechanical');
#15180=PRODUCT('Base','Base','Base',(#15177));
#15257=COLOUR_RGB('Dark Blue',0.08,0.2,0.34);
#15258=FILL_AREA_STYLE_COLOUR('',#15257);
#15259=FILL_AREA_STYLE('',(#15258));
#15260=SURFACE_STYLE_FILL_AREA(#15259);
#15261=SURFACE_SIDE_STYLE('',(#15260));
#15262=SURFACE_STYLE_USAGE(.BOTH.,#15261);
#15263=PRESENTATION_STYLE_ASSIGNMENT((#15262));
ENDSEC;
END-ISO-10303-21;
